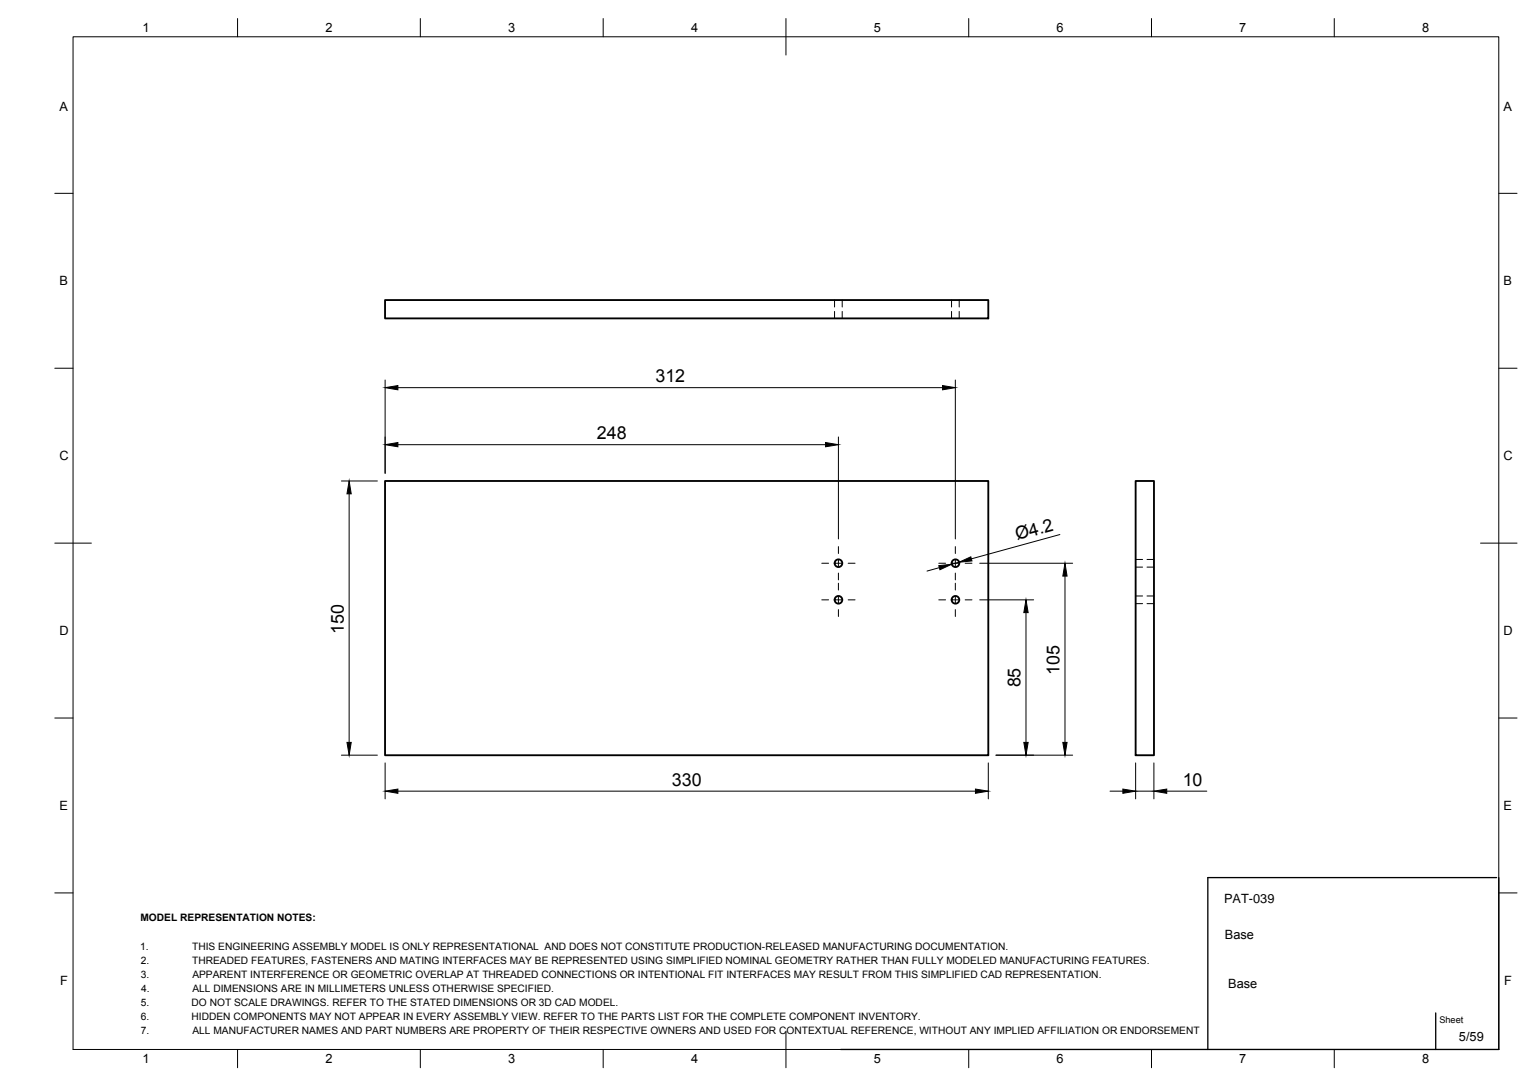
ISO-10303-21;
HEADER;
/* Generated by software containing ST-Developer
 * from STEP Tools, Inc. (www.steptools.com) 
 */

FILE_DESCRIPTION(
/* description */ ('Four-bar parallelogram arm'),
/* implementation_level */ '2;1');

FILE_NAME(
/* name */ 'Base.step',
/* time_stamp */ '2026-10-28T03:24:55-07:00',
/* author */ (''),
/* organization */ (''),
/* preprocessor_version */ 'ST-DEVELOPER v20.2',
/* originating_system */ 'Autodesk Translation Framework v15.17.0.0',
/* authorisation */ '');

FILE_SCHEMA (('AUTOMOTIVE_DESIGN { 1 0 10303 214 3 1 1 }'));
ENDSEC;

DATA;
#10=MECHANICAL_DESIGN_GEOMETRIC_PRESENTATION_REPRESENTATION('',(#622),#14512);
#522=SHAPE_REPRESENTATION_RELATIONSHIP('SRR','None',#14743,#572);
#572=ADVANCED_BREP_SHAPE_REPRESENTATION('',(#680),#14458);
#622=STYLED_ITEM('',(#15066),#680);
#680=MANIFOLD_SOLID_BREP('Body1',#7326);
#735=FACE_BOUND('',#1630,.T.);
#736=FACE_BOUND('',#1631,.T.);
#737=FACE_BOUND('',#1632,.T.);
#738=FACE_BOUND('',#1633,.T.);
#739=FACE_BOUND('',#1635,.T.);
#740=FACE_BOUND('',#1636,.T.);
#741=FACE_BOUND('',#1637,.T.);
#742=FACE_BOUND('',#1638,.T.);
#1006=PLANE('',#7953);
#1007=PLANE('',#7954);
#1008=PLANE('',#7955);
#1009=PLANE('',#7956);
#1010=PLANE('',#7957);
#1011=PLANE('',#7958);
#1201=FACE_OUTER_BOUND('',#1621,.T.);
#1202=FACE_OUTER_BOUND('',#1622,.T.);
#1203=FACE_OUTER_BOUND('',#1623,.T.);
#1204=FACE_OUTER_BOUND('',#1624,.T.);
#1205=FACE_OUTER_BOUND('',#1625,.T.);
#1206=FACE_OUTER_BOUND('',#1626,.T.);
#1207=FACE_OUTER_BOUND('',#1627,.T.);
#1208=FACE_OUTER_BOUND('',#1628,.T.);
#1209=FACE_OUTER_BOUND('',#1629,.T.);
#1210=FACE_OUTER_BOUND('',#1634,.T.);
#1621=EDGE_LOOP('',(#4988,#4989,#4990,#4991));
#1622=EDGE_LOOP('',(#4992,#4993,#4994,#4995));
#1623=EDGE_LOOP('',(#4996,#4997,#4998,#4999));
#1624=EDGE_LOOP('',(#5000,#5001,#5002,#5003));
#1625=EDGE_LOOP('',(#5004,#5005,#5006,#5007));
#1626=EDGE_LOOP('',(#5008,#5009,#5010,#5011));
#1627=EDGE_LOOP('',(#5012,#5013,#5014,#5015));
#1628=EDGE_LOOP('',(#5016,#5017,#5018,#5019));
#1629=EDGE_LOOP('',(#5020,#5021,#5022,#5023));
#1630=EDGE_LOOP('',(#5024));
#1631=EDGE_LOOP('',(#5025));
#1632=EDGE_LOOP('',(#5026));
#1633=EDGE_LOOP('',(#5027));
#1634=EDGE_LOOP('',(#5028,#5029,#5030,#5031));
#1635=EDGE_LOOP('',(#5032));
#1636=EDGE_LOOP('',(#5033));
#1637=EDGE_LOOP('',(#5034));
#1638=EDGE_LOOP('',(#5035));
#2312=LINE('',#11435,#2706);
#2313=LINE('',#11441,#2707);
#2314=LINE('',#11447,#2708);
#2315=LINE('',#11453,#2709);
#2316=LINE('',#11458,#2710);
#2317=LINE('',#11460,#2711);
#2318=LINE('',#11462,#2712);
#2319=LINE('',#11463,#2713);
#2320=LINE('',#11466,#2714);
#2321=LINE('',#11468,#2715);
#2322=LINE('',#11469,#2716);
#2323=LINE('',#11472,#2717);
#2324=LINE('',#11474,#2718);
#2325=LINE('',#11475,#2719);
#2326=LINE('',#11477,#2720);
#2327=LINE('',#11478,#2721);
#2706=VECTOR('',#8980,0.21);
#2707=VECTOR('',#8987,0.21);
#2708=VECTOR('',#8994,0.21);
#2709=VECTOR('',#9001,0.21);
#2710=VECTOR('',#9006,1.);
#2711=VECTOR('',#9007,1.);
#2712=VECTOR('',#9008,1.);
#2713=VECTOR('',#9009,1.);
#2714=VECTOR('',#9012,1.);
#2715=VECTOR('',#9013,1.);
#2716=VECTOR('',#9014,1.);
#2717=VECTOR('',#9017,1.);
#2718=VECTOR('',#9018,1.);
#2719=VECTOR('',#9019,1.);
#2720=VECTOR('',#9022,1.);
#2721=VECTOR('',#9023,1.);
#3100=CIRCLE('',#7942,0.21);
#3101=CIRCLE('',#7943,0.21);
#3102=CIRCLE('',#7945,0.21);
#3103=CIRCLE('',#7946,0.21);
#3104=CIRCLE('',#7948,0.21);
#3105=CIRCLE('',#7949,0.21);
#3106=CIRCLE('',#7951,0.21);
#3107=CIRCLE('',#7952,0.21);
#3545=VERTEX_POINT('',#11432);
#3546=VERTEX_POINT('',#11434);
#3547=VERTEX_POINT('',#11438);
#3548=VERTEX_POINT('',#11440);
#3549=VERTEX_POINT('',#11444);
#3550=VERTEX_POINT('',#11446);
#3551=VERTEX_POINT('',#11450);
#3552=VERTEX_POINT('',#11452);
#3553=VERTEX_POINT('',#11456);
#3554=VERTEX_POINT('',#11457);
#3555=VERTEX_POINT('',#11459);
#3556=VERTEX_POINT('',#11461);
#3557=VERTEX_POINT('',#11465);
#3558=VERTEX_POINT('',#11467);
#3559=VERTEX_POINT('',#11471);
#3560=VERTEX_POINT('',#11473);
#4125=EDGE_CURVE('',#3545,#3545,#3100,.T.);
#4126=EDGE_CURVE('',#3545,#3546,#2312,.T.);
#4127=EDGE_CURVE('',#3546,#3546,#3101,.T.);
#4128=EDGE_CURVE('',#3547,#3547,#3102,.T.);
#4129=EDGE_CURVE('',#3547,#3548,#2313,.T.);
#4130=EDGE_CURVE('',#3548,#3548,#3103,.T.);
#4131=EDGE_CURVE('',#3549,#3549,#3104,.T.);
#4132=EDGE_CURVE('',#3549,#3550,#2314,.T.);
#4133=EDGE_CURVE('',#3550,#3550,#3105,.T.);
#4134=EDGE_CURVE('',#3551,#3551,#3106,.T.);
#4135=EDGE_CURVE('',#3551,#3552,#2315,.T.);
#4136=EDGE_CURVE('',#3552,#3552,#3107,.T.);
#4137=EDGE_CURVE('',#3553,#3554,#2316,.T.);
#4138=EDGE_CURVE('',#3554,#3555,#2317,.T.);
#4139=EDGE_CURVE('',#3556,#3555,#2318,.T.);
#4140=EDGE_CURVE('',#3553,#3556,#2319,.T.);
#4141=EDGE_CURVE('',#3557,#3553,#2320,.T.);
#4142=EDGE_CURVE('',#3558,#3556,#2321,.T.);
#4143=EDGE_CURVE('',#3557,#3558,#2322,.T.);
#4144=EDGE_CURVE('',#3559,#3557,#2323,.T.);
#4145=EDGE_CURVE('',#3560,#3558,#2324,.T.);
#4146=EDGE_CURVE('',#3559,#3560,#2325,.T.);
#4147=EDGE_CURVE('',#3554,#3559,#2326,.T.);
#4148=EDGE_CURVE('',#3555,#3560,#2327,.T.);
#4988=ORIENTED_EDGE('',*,*,#4125,.F.);
#4989=ORIENTED_EDGE('',*,*,#4126,.T.);
#4990=ORIENTED_EDGE('',*,*,#4127,.F.);
#4991=ORIENTED_EDGE('',*,*,#4126,.F.);
#4992=ORIENTED_EDGE('',*,*,#4128,.F.);
#4993=ORIENTED_EDGE('',*,*,#4129,.T.);
#4994=ORIENTED_EDGE('',*,*,#4130,.F.);
#4995=ORIENTED_EDGE('',*,*,#4129,.F.);
#4996=ORIENTED_EDGE('',*,*,#4131,.F.);
#4997=ORIENTED_EDGE('',*,*,#4132,.T.);
#4998=ORIENTED_EDGE('',*,*,#4133,.F.);
#4999=ORIENTED_EDGE('',*,*,#4132,.F.);
#5000=ORIENTED_EDGE('',*,*,#4134,.F.);
#5001=ORIENTED_EDGE('',*,*,#4135,.T.);
#5002=ORIENTED_EDGE('',*,*,#4136,.F.);
#5003=ORIENTED_EDGE('',*,*,#4135,.F.);
#5004=ORIENTED_EDGE('',*,*,#4137,.T.);
#5005=ORIENTED_EDGE('',*,*,#4138,.T.);
#5006=ORIENTED_EDGE('',*,*,#4139,.F.);
#5007=ORIENTED_EDGE('',*,*,#4140,.F.);
#5008=ORIENTED_EDGE('',*,*,#4141,.T.);
#5009=ORIENTED_EDGE('',*,*,#4140,.T.);
#5010=ORIENTED_EDGE('',*,*,#4142,.F.);
#5011=ORIENTED_EDGE('',*,*,#4143,.F.);
#5012=ORIENTED_EDGE('',*,*,#4144,.T.);
#5013=ORIENTED_EDGE('',*,*,#4143,.T.);
#5014=ORIENTED_EDGE('',*,*,#4145,.F.);
#5015=ORIENTED_EDGE('',*,*,#4146,.F.);
#5016=ORIENTED_EDGE('',*,*,#4147,.T.);
#5017=ORIENTED_EDGE('',*,*,#4146,.T.);
#5018=ORIENTED_EDGE('',*,*,#4148,.F.);
#5019=ORIENTED_EDGE('',*,*,#4138,.F.);
#5020=ORIENTED_EDGE('',*,*,#4148,.T.);
#5021=ORIENTED_EDGE('',*,*,#4145,.T.);
#5022=ORIENTED_EDGE('',*,*,#4142,.T.);
#5023=ORIENTED_EDGE('',*,*,#4139,.T.);
#5024=ORIENTED_EDGE('',*,*,#4127,.T.);
#5025=ORIENTED_EDGE('',*,*,#4130,.T.);
#5026=ORIENTED_EDGE('',*,*,#4133,.T.);
#5027=ORIENTED_EDGE('',*,*,#4136,.T.);
#5028=ORIENTED_EDGE('',*,*,#4147,.F.);
#5029=ORIENTED_EDGE('',*,*,#4137,.F.);
#5030=ORIENTED_EDGE('',*,*,#4141,.F.);
#5031=ORIENTED_EDGE('',*,*,#4144,.F.);
#5032=ORIENTED_EDGE('',*,*,#4125,.T.);
#5033=ORIENTED_EDGE('',*,*,#4128,.T.);
#5034=ORIENTED_EDGE('',*,*,#4131,.T.);
#5035=ORIENTED_EDGE('',*,*,#4134,.T.);
#6714=CYLINDRICAL_SURFACE('',#7941,0.21);
#6715=CYLINDRICAL_SURFACE('',#7944,0.21);
#6716=CYLINDRICAL_SURFACE('',#7947,0.21);
#6717=CYLINDRICAL_SURFACE('',#7950,0.21);
#6906=ADVANCED_FACE('',(#1201),#6714,.F.);
#6907=ADVANCED_FACE('',(#1202),#6715,.F.);
#6908=ADVANCED_FACE('',(#1203),#6716,.F.);
#6909=ADVANCED_FACE('',(#1204),#6717,.F.);
#6910=ADVANCED_FACE('',(#1205),#1006,.T.);
#6911=ADVANCED_FACE('',(#1206),#1007,.T.);
#6912=ADVANCED_FACE('',(#1207),#1008,.T.);
#6913=ADVANCED_FACE('',(#1208),#1009,.T.);
#6914=ADVANCED_FACE('',(#1209,#735,#736,#737,#738),#1010,.T.);
#6915=ADVANCED_FACE('',(#1210,#739,#740,#741,#742),#1011,.F.);
#7326=CLOSED_SHELL('',(#6906,#6907,#6908,#6909,#6910,#6911,#6912,#6913,
#6914,#6915));
#7940=AXIS2_PLACEMENT_3D('',#11430,#8974,#8975);
#7941=AXIS2_PLACEMENT_3D('',#11431,#8976,#8977);
#7942=AXIS2_PLACEMENT_3D('',#11433,#8978,#8979);
#7943=AXIS2_PLACEMENT_3D('',#11436,#8981,#8982);
#7944=AXIS2_PLACEMENT_3D('',#11437,#8983,#8984);
#7945=AXIS2_PLACEMENT_3D('',#11439,#8985,#8986);
#7946=AXIS2_PLACEMENT_3D('',#11442,#8988,#8989);
#7947=AXIS2_PLACEMENT_3D('',#11443,#8990,#8991);
#7948=AXIS2_PLACEMENT_3D('',#11445,#8992,#8993);
#7949=AXIS2_PLACEMENT_3D('',#11448,#8995,#8996);
#7950=AXIS2_PLACEMENT_3D('',#11449,#8997,#8998);
#7951=AXIS2_PLACEMENT_3D('',#11451,#8999,#9000);
#7952=AXIS2_PLACEMENT_3D('',#11454,#9002,#9003);
#7953=AXIS2_PLACEMENT_3D('',#11455,#9004,#9005);
#7954=AXIS2_PLACEMENT_3D('',#11464,#9010,#9011);
#7955=AXIS2_PLACEMENT_3D('',#11470,#9015,#9016);
#7956=AXIS2_PLACEMENT_3D('',#11476,#9020,#9021);
#7957=AXIS2_PLACEMENT_3D('',#11479,#9024,#9025);
#7958=AXIS2_PLACEMENT_3D('',#11480,#9026,#9027);
#8974=DIRECTION('axis',(0.,0.,1.));
#8975=DIRECTION('refdir',(1.,0.,0.));
#8976=DIRECTION('center_axis',(0.,0.,1.));
#8977=DIRECTION('ref_axis',(1.,0.,0.));
#8978=DIRECTION('center_axis',(0.,0.,1.));
#8979=DIRECTION('ref_axis',(1.,0.,0.));
#8980=DIRECTION('',(0.,0.,1.));
#8981=DIRECTION('center_axis',(0.,0.,-1.));
#8982=DIRECTION('ref_axis',(1.,0.,0.));
#8983=DIRECTION('center_axis',(0.,0.,1.));
#8984=DIRECTION('ref_axis',(1.,0.,0.));
#8985=DIRECTION('center_axis',(0.,0.,1.));
#8986=DIRECTION('ref_axis',(1.,0.,0.));
#8987=DIRECTION('',(0.,0.,1.));
#8988=DIRECTION('center_axis',(0.,0.,-1.));
#8989=DIRECTION('ref_axis',(1.,0.,0.));
#8990=DIRECTION('center_axis',(0.,0.,1.));
#8991=DIRECTION('ref_axis',(1.,0.,0.));
#8992=DIRECTION('center_axis',(0.,0.,1.));
#8993=DIRECTION('ref_axis',(1.,0.,0.));
#8994=DIRECTION('',(0.,0.,1.));
#8995=DIRECTION('center_axis',(0.,0.,-1.));
#8996=DIRECTION('ref_axis',(1.,0.,0.));
#8997=DIRECTION('center_axis',(0.,0.,1.));
#8998=DIRECTION('ref_axis',(1.,0.,0.));
#8999=DIRECTION('center_axis',(0.,0.,1.));
#9000=DIRECTION('ref_axis',(1.,0.,0.));
#9001=DIRECTION('',(0.,0.,1.));
#9002=DIRECTION('center_axis',(0.,0.,-1.));
#9003=DIRECTION('ref_axis',(1.,0.,0.));
#9004=DIRECTION('center_axis',(0.,1.,0.));
#9005=DIRECTION('ref_axis',(-1.,0.,0.));
#9006=DIRECTION('',(-1.,0.,0.));
#9007=DIRECTION('',(0.,0.,1.));
#9008=DIRECTION('',(-1.,0.,0.));
#9009=DIRECTION('',(0.,0.,1.));
#9010=DIRECTION('center_axis',(1.,0.,0.));
#9011=DIRECTION('ref_axis',(0.,1.,0.));
#9012=DIRECTION('',(0.,1.,0.));
#9013=DIRECTION('',(0.,1.,0.));
#9014=DIRECTION('',(0.,0.,1.));
#9015=DIRECTION('center_axis',(0.,-1.,0.));
#9016=DIRECTION('ref_axis',(1.,0.,0.));
#9017=DIRECTION('',(1.,0.,0.));
#9018=DIRECTION('',(1.,0.,0.));
#9019=DIRECTION('',(0.,0.,1.));
#9020=DIRECTION('center_axis',(-1.,0.,0.));
#9021=DIRECTION('ref_axis',(0.,-1.,0.));
#9022=DIRECTION('',(0.,-1.,0.));
#9023=DIRECTION('',(0.,-1.,0.));
#9024=DIRECTION('center_axis',(0.,0.,1.));
#9025=DIRECTION('ref_axis',(1.,0.,0.));
#9026=DIRECTION('center_axis',(0.,0.,1.));
#9027=DIRECTION('ref_axis',(1.,0.,0.));
#11430=CARTESIAN_POINT('',(0.,0.,0.));
#11431=CARTESIAN_POINT('Origin',(3.2,3.5,-0.1));
#11432=CARTESIAN_POINT('',(2.99,3.5,0.));
#11433=CARTESIAN_POINT('Origin',(3.2,3.5,0.));
#11434=CARTESIAN_POINT('',(2.99,3.5,1.));
#11435=CARTESIAN_POINT('',(2.99,3.5,-0.1));
#11436=CARTESIAN_POINT('Origin',(3.2,3.5,1.));
#11437=CARTESIAN_POINT('Origin',(-3.2,5.5,-0.1));
#11438=CARTESIAN_POINT('',(-3.41,5.5,0.));
#11439=CARTESIAN_POINT('Origin',(-3.2,5.5,0.));
#11440=CARTESIAN_POINT('',(-3.41,5.5,1.));
#11441=CARTESIAN_POINT('',(-3.41,5.5,-0.1));
#11442=CARTESIAN_POINT('Origin',(-3.2,5.5,1.));
#11443=CARTESIAN_POINT('Origin',(-3.2,3.5,-0.1));
#11444=CARTESIAN_POINT('',(-3.41,3.5,0.));
#11445=CARTESIAN_POINT('Origin',(-3.2,3.5,0.));
#11446=CARTESIAN_POINT('',(-3.41,3.5,1.));
#11447=CARTESIAN_POINT('',(-3.41,3.5,-0.1));
#11448=CARTESIAN_POINT('Origin',(-3.2,3.5,1.));
#11449=CARTESIAN_POINT('Origin',(3.2,5.5,-0.1));
#11450=CARTESIAN_POINT('',(2.99,5.5,0.));
#11451=CARTESIAN_POINT('Origin',(3.2,5.5,0.));
#11452=CARTESIAN_POINT('',(2.99,5.5,1.));
#11453=CARTESIAN_POINT('',(2.99,5.5,-0.1));
#11454=CARTESIAN_POINT('Origin',(3.2,5.5,1.));
#11455=CARTESIAN_POINT('Origin',(28.,10.,0.));
#11456=CARTESIAN_POINT('',(28.,10.,0.));
#11457=CARTESIAN_POINT('',(-5.,10.,0.));
#11458=CARTESIAN_POINT('',(28.,10.,0.));
#11459=CARTESIAN_POINT('',(-5.,10.,1.));
#11460=CARTESIAN_POINT('',(-5.,10.,0.));
#11461=CARTESIAN_POINT('',(28.,10.,1.));
#11462=CARTESIAN_POINT('',(28.,10.,1.));
#11463=CARTESIAN_POINT('',(28.,10.,0.));
#11464=CARTESIAN_POINT('Origin',(28.,-5.,0.));
#11465=CARTESIAN_POINT('',(28.,-5.,0.));
#11466=CARTESIAN_POINT('',(28.,-5.,0.));
#11467=CARTESIAN_POINT('',(28.,-5.,1.));
#11468=CARTESIAN_POINT('',(28.,-5.,1.));
#11469=CARTESIAN_POINT('',(28.,-5.,0.));
#11470=CARTESIAN_POINT('Origin',(-5.,-5.,0.));
#11471=CARTESIAN_POINT('',(-5.,-5.,0.));
#11472=CARTESIAN_POINT('',(-5.,-5.,0.));
#11473=CARTESIAN_POINT('',(-5.,-5.,1.));
#11474=CARTESIAN_POINT('',(-5.,-5.,1.));
#11475=CARTESIAN_POINT('',(-5.,-5.,0.));
#11476=CARTESIAN_POINT('Origin',(-5.,10.,0.));
#11477=CARTESIAN_POINT('',(-5.,10.,0.));
#11478=CARTESIAN_POINT('',(-5.,10.,1.));
#11479=CARTESIAN_POINT('Origin',(11.5,2.5,1.));
#11480=CARTESIAN_POINT('Origin',(11.5,2.5,0.));
#14401=UNCERTAINTY_MEASURE_WITH_UNIT(LENGTH_MEASURE(0.001),#14513,
'DISTANCE_ACCURACY_VALUE',
'Maximum model space distance between geometric entities at asserted c
onnectivities');
#14455=UNCERTAINTY_MEASURE_WITH_UNIT(LENGTH_MEASURE(0.001),#14513,
'DISTANCE_ACCURACY_VALUE',
'Maximum model space distance between geometric entities at asserted c
onnectivities');
#14458=(
GEOMETRIC_REPRESENTATION_CONTEXT(3)
GLOBAL_UNCERTAINTY_ASSIGNED_CONTEXT((#14401))
GLOBAL_UNIT_ASSIGNED_CONTEXT((#14513,#14515,#14516))
REPRESENTATION_CONTEXT('','3D')
);
#14512=(
GEOMETRIC_REPRESENTATION_CONTEXT(3)
GLOBAL_UNCERTAINTY_ASSIGNED_CONTEXT((#14455))
GLOBAL_UNIT_ASSIGNED_CONTEXT((#14513,#14515,#14516))
REPRESENTATION_CONTEXT('','3D')
);
#14513=(
LENGTH_UNIT()
NAMED_UNIT(*)
SI_UNIT(.CENTI.,.METRE.)
);
#14515=(
NAMED_UNIT(*)
PLANE_ANGLE_UNIT()
SI_UNIT($,.RADIAN.)
);
#14516=(
NAMED_UNIT(*)
SI_UNIT($,.STERADIAN.)
SOLID_ANGLE_UNIT()
);
#14519=SHAPE_DEFINITION_REPRESENTATION(#14575,#14743);
#14575=PRODUCT_DEFINITION_SHAPE('',$,#14800);
#14743=SHAPE_REPRESENTATION('',(#7940),#14458);
#14797=PRODUCT_DEFINITION_CONTEXT('part definition',#14967,'design');
#14800=PRODUCT_DEFINITION('Base','Base',#14856,#14797);
#14856=PRODUCT_DEFINITION_FORMATION('',$,#14971);
#14967=APPLICATION_CONTEXT(
'Core Data for Automotive Mechanical Design Process');
#14968=PRODUCT_CONTEXT('part definition',#14967,'mechanical');
#14971=PRODUCT('Base','Base','Base',(#14968));
#15060=COLOUR_RGB('Dark Blue',0.08,0.2,0.34);
#15061=FILL_AREA_STYLE_COLOUR('',#15060);
#15062=FILL_AREA_STYLE('',(#15061));
#15063=SURFACE_STYLE_FILL_AREA(#15062);
#15064=SURFACE_SIDE_STYLE('',(#15063));
#15065=SURFACE_STYLE_USAGE(.BOTH.,#15064);
#15066=PRESENTATION_STYLE_ASSIGNMENT((#15065));
ENDSEC;
END-ISO-10303-21;
